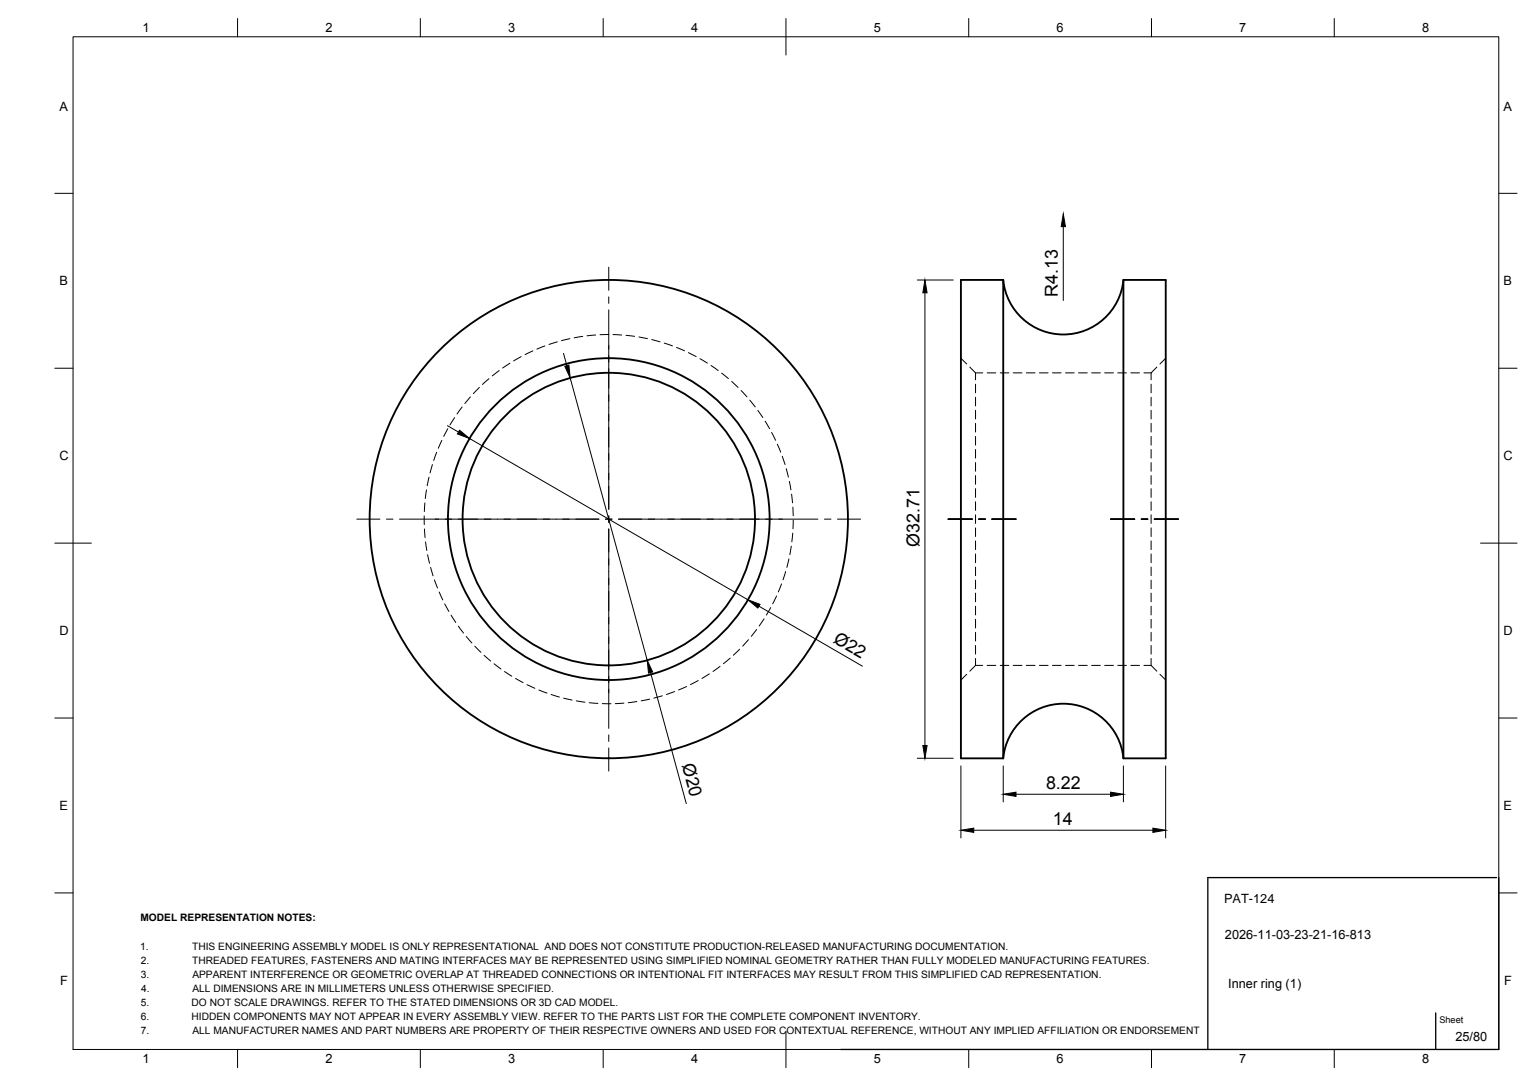
ISO-10303-21;
HEADER;
/* Generated by software containing ST-Developer
 * from STEP Tools, Inc. (www.steptools.com) 
 */

FILE_DESCRIPTION(
/* description */ ('XY cross-slide table'),
/* implementation_level */ '2;1');

FILE_NAME(
/* name */ 'Inner ring (1).step',
/* time_stamp */ '2026-10-28T03:22:46-07:00',
/* author */ (''),
/* organization */ (''),
/* preprocessor_version */ 'ST-DEVELOPER v20.2',
/* originating_system */ 'Autodesk Translation Framework v15.17.0.0',
/* authorisation */ '');

FILE_SCHEMA (('AUTOMOTIVE_DESIGN { 1 0 10303 214 3 1 1 }'));
ENDSEC;

DATA;
#10=MECHANICAL_DESIGN_GEOMETRIC_PRESENTATION_REPRESENTATION('',(#1693),#62984);
#1445=CONICAL_SURFACE('',#24426,1.05,0.785398163397449);
#1446=CONICAL_SURFACE('',#24433,1.05,0.785398163397449);
#1498=TOROIDAL_SURFACE('',#24415,1.675,0.412776);
#1520=SHAPE_REPRESENTATION_RELATIONSHIP('SRR','None',#63370,#1603);
#1603=ADVANCED_BREP_SHAPE_REPRESENTATION('',(#1806),#62907);
#1693=STYLED_ITEM('',(#63912),#1806);
#1806=MANIFOLD_SOLID_BREP('Body1',#22987);
#1992=FACE_BOUND('',#4488,.T.);
#1993=FACE_BOUND('',#4491,.T.);
#2397=PLANE('',#24428);
#2398=PLANE('',#24431);
#3064=FACE_OUTER_BOUND('',#4483,.T.);
#3065=FACE_OUTER_BOUND('',#4484,.T.);
#3066=FACE_OUTER_BOUND('',#4485,.T.);
#3067=FACE_OUTER_BOUND('',#4486,.T.);
#3068=FACE_OUTER_BOUND('',#4487,.T.);
#3069=FACE_OUTER_BOUND('',#4489,.T.);
#3070=FACE_OUTER_BOUND('',#4490,.T.);
#3071=FACE_OUTER_BOUND('',#4492,.T.);
#4483=EDGE_LOOP('',(#15752,#15753,#15754,#15755,#15756,#15757));
#4484=EDGE_LOOP('',(#15758,#15759,#15760,#15761,#15762));
#4485=EDGE_LOOP('',(#15763,#15764,#15765,#15766));
#4486=EDGE_LOOP('',(#15767,#15768,#15769,#15770));
#4487=EDGE_LOOP('',(#15771));
#4488=EDGE_LOOP('',(#15772));
#4489=EDGE_LOOP('',(#15773,#15774,#15775,#15776,#15777));
#4490=EDGE_LOOP('',(#15778));
#4491=EDGE_LOOP('',(#15779));
#4492=EDGE_LOOP('',(#15780,#15781,#15782,#15783));
#6123=LINE('',#34110,#7610);
#6124=LINE('',#34116,#7611);
#6125=LINE('',#34120,#7612);
#6126=LINE('',#34126,#7613);
#6127=LINE('',#34131,#7614);
#7610=VECTOR('',#27522,1.63531);
#7611=VECTOR('',#27529,1.);
#7612=VECTOR('',#27534,1.05);
#7613=VECTOR('',#27543,1.63531);
#7614=VECTOR('',#27550,1.05);
#9073=CIRCLE('',#24416,1.63531);
#9074=CIRCLE('',#24417,1.63531);
#9075=CIRCLE('',#24418,0.412776);
#9076=CIRCLE('',#24419,1.63531);
#9077=CIRCLE('',#24420,1.63531);
#9078=CIRCLE('',#24422,1.63531);
#9079=CIRCLE('',#24424,1.);
#9080=CIRCLE('',#24425,1.);
#9081=CIRCLE('',#24427,1.1);
#9082=CIRCLE('',#24430,1.63531);
#9083=CIRCLE('',#24432,1.1);
#10061=VERTEX_POINT('',#34099);
#10062=VERTEX_POINT('',#34100);
#10063=VERTEX_POINT('',#34103);
#10064=VERTEX_POINT('',#34105);
#10065=VERTEX_POINT('',#34109);
#10066=VERTEX_POINT('',#34113);
#10067=VERTEX_POINT('',#34115);
#10068=VERTEX_POINT('',#34119);
#10069=VERTEX_POINT('',#34124);
#10070=VERTEX_POINT('',#34128);
#12260=EDGE_CURVE('',#10061,#10062,#9073,.T.);
#12261=EDGE_CURVE('',#10062,#10061,#9074,.T.);
#12262=EDGE_CURVE('',#10062,#10063,#9075,.T.);
#12263=EDGE_CURVE('',#10064,#10063,#9076,.T.);
#12264=EDGE_CURVE('',#10063,#10064,#9077,.T.);
#12265=EDGE_CURVE('',#10064,#10065,#6123,.T.);
#12266=EDGE_CURVE('',#10065,#10065,#9078,.T.);
#12267=EDGE_CURVE('',#10066,#10066,#9079,.T.);
#12268=EDGE_CURVE('',#10066,#10067,#6124,.T.);
#12269=EDGE_CURVE('',#10067,#10067,#9080,.T.);
#12270=EDGE_CURVE('',#10067,#10068,#6125,.T.);
#12271=EDGE_CURVE('',#10068,#10068,#9081,.T.);
#12272=EDGE_CURVE('',#10069,#10069,#9082,.T.);
#12273=EDGE_CURVE('',#10069,#10061,#6126,.T.);
#12274=EDGE_CURVE('',#10070,#10070,#9083,.T.);
#12275=EDGE_CURVE('',#10070,#10066,#6127,.T.);
#15752=ORIENTED_EDGE('',*,*,#12260,.F.);
#15753=ORIENTED_EDGE('',*,*,#12261,.F.);
#15754=ORIENTED_EDGE('',*,*,#12262,.T.);
#15755=ORIENTED_EDGE('',*,*,#12263,.F.);
#15756=ORIENTED_EDGE('',*,*,#12264,.F.);
#15757=ORIENTED_EDGE('',*,*,#12262,.F.);
#15758=ORIENTED_EDGE('',*,*,#12263,.T.);
#15759=ORIENTED_EDGE('',*,*,#12264,.T.);
#15760=ORIENTED_EDGE('',*,*,#12265,.T.);
#15761=ORIENTED_EDGE('',*,*,#12266,.T.);
#15762=ORIENTED_EDGE('',*,*,#12265,.F.);
#15763=ORIENTED_EDGE('',*,*,#12267,.T.);
#15764=ORIENTED_EDGE('',*,*,#12268,.T.);
#15765=ORIENTED_EDGE('',*,*,#12269,.F.);
#15766=ORIENTED_EDGE('',*,*,#12268,.F.);
#15767=ORIENTED_EDGE('',*,*,#12269,.T.);
#15768=ORIENTED_EDGE('',*,*,#12270,.T.);
#15769=ORIENTED_EDGE('',*,*,#12271,.F.);
#15770=ORIENTED_EDGE('',*,*,#12270,.F.);
#15771=ORIENTED_EDGE('',*,*,#12266,.F.);
#15772=ORIENTED_EDGE('',*,*,#12271,.T.);
#15773=ORIENTED_EDGE('',*,*,#12272,.F.);
#15774=ORIENTED_EDGE('',*,*,#12273,.T.);
#15775=ORIENTED_EDGE('',*,*,#12260,.T.);
#15776=ORIENTED_EDGE('',*,*,#12261,.T.);
#15777=ORIENTED_EDGE('',*,*,#12273,.F.);
#15778=ORIENTED_EDGE('',*,*,#12272,.T.);
#15779=ORIENTED_EDGE('',*,*,#12274,.F.);
#15780=ORIENTED_EDGE('',*,*,#12274,.T.);
#15781=ORIENTED_EDGE('',*,*,#12275,.T.);
#15782=ORIENTED_EDGE('',*,*,#12267,.F.);
#15783=ORIENTED_EDGE('',*,*,#12275,.F.);
#21114=CYLINDRICAL_SURFACE('',#24421,1.63531);
#21115=CYLINDRICAL_SURFACE('',#24423,1.);
#21116=CYLINDRICAL_SURFACE('',#24429,1.63531);
#21845=ADVANCED_FACE('',(#3064),#1498,.F.);
#21846=ADVANCED_FACE('',(#3065),#21114,.T.);
#21847=ADVANCED_FACE('',(#3066),#21115,.F.);
#21848=ADVANCED_FACE('',(#3067),#1445,.F.);
#21849=ADVANCED_FACE('',(#3068,#1992),#2397,.T.);
#21850=ADVANCED_FACE('',(#3069),#21116,.T.);
#21851=ADVANCED_FACE('',(#3070,#1993),#2398,.T.);
#21852=ADVANCED_FACE('',(#3071),#1446,.F.);
#22987=CLOSED_SHELL('',(#21845,#21846,#21847,#21848,#21849,#21850,#21851,
#21852));
#24414=AXIS2_PLACEMENT_3D('',#34097,#27506,#27507);
#24415=AXIS2_PLACEMENT_3D('',#34098,#27508,#27509);
#24416=AXIS2_PLACEMENT_3D('',#34101,#27510,#27511);
#24417=AXIS2_PLACEMENT_3D('',#34102,#27512,#27513);
#24418=AXIS2_PLACEMENT_3D('',#34104,#27514,#27515);
#24419=AXIS2_PLACEMENT_3D('',#34106,#27516,#27517);
#24420=AXIS2_PLACEMENT_3D('',#34107,#27518,#27519);
#24421=AXIS2_PLACEMENT_3D('',#34108,#27520,#27521);
#24422=AXIS2_PLACEMENT_3D('',#34111,#27523,#27524);
#24423=AXIS2_PLACEMENT_3D('',#34112,#27525,#27526);
#24424=AXIS2_PLACEMENT_3D('',#34114,#27527,#27528);
#24425=AXIS2_PLACEMENT_3D('',#34117,#27530,#27531);
#24426=AXIS2_PLACEMENT_3D('',#34118,#27532,#27533);
#24427=AXIS2_PLACEMENT_3D('',#34121,#27535,#27536);
#24428=AXIS2_PLACEMENT_3D('',#34122,#27537,#27538);
#24429=AXIS2_PLACEMENT_3D('',#34123,#27539,#27540);
#24430=AXIS2_PLACEMENT_3D('',#34125,#27541,#27542);
#24431=AXIS2_PLACEMENT_3D('',#34127,#27544,#27545);
#24432=AXIS2_PLACEMENT_3D('',#34129,#27546,#27547);
#24433=AXIS2_PLACEMENT_3D('',#34130,#27548,#27549);
#27506=DIRECTION('axis',(0.,0.,1.));
#27507=DIRECTION('refdir',(1.,0.,0.));
#27508=DIRECTION('center_axis',(0.,-1.,0.));
#27509=DIRECTION('ref_axis',(0.,0.,-1.));
#27510=DIRECTION('center_axis',(0.,-1.,0.));
#27511=DIRECTION('ref_axis',(1.,0.,0.));
#27512=DIRECTION('center_axis',(0.,-1.,0.));
#27513=DIRECTION('ref_axis',(1.,0.,0.));
#27514=DIRECTION('center_axis',(1.,0.,1.22464679914735E-16));
#27515=DIRECTION('ref_axis',(-1.22464679914735E-16,0.,1.));
#27516=DIRECTION('center_axis',(0.,1.,0.));
#27517=DIRECTION('ref_axis',(1.,0.,0.));
#27518=DIRECTION('center_axis',(0.,1.,0.));
#27519=DIRECTION('ref_axis',(1.,0.,0.));
#27520=DIRECTION('center_axis',(0.,-1.,0.));
#27521=DIRECTION('ref_axis',(1.,0.,0.));
#27522=DIRECTION('',(0.,1.,0.));
#27523=DIRECTION('center_axis',(0.,-1.,0.));
#27524=DIRECTION('ref_axis',(1.,0.,0.));
#27525=DIRECTION('center_axis',(0.,-1.,0.));
#27526=DIRECTION('ref_axis',(1.,0.,0.));
#27527=DIRECTION('center_axis',(0.,-1.,0.));
#27528=DIRECTION('ref_axis',(1.,0.,0.));
#27529=DIRECTION('',(0.,1.,0.));
#27530=DIRECTION('center_axis',(0.,-1.,0.));
#27531=DIRECTION('ref_axis',(1.,0.,0.));
#27532=DIRECTION('center_axis',(0.,1.,0.));
#27533=DIRECTION('ref_axis',(1.,0.,0.));
#27534=DIRECTION('',(-0.707106781186548,0.707106781186547,-8.65956056235494E-17));
#27535=DIRECTION('center_axis',(0.,-1.,0.));
#27536=DIRECTION('ref_axis',(1.,0.,0.));
#27537=DIRECTION('center_axis',(0.,1.,0.));
#27538=DIRECTION('ref_axis',(0.,0.,1.));
#27539=DIRECTION('center_axis',(0.,-1.,0.));
#27540=DIRECTION('ref_axis',(1.,0.,0.));
#27541=DIRECTION('center_axis',(0.,-1.,0.));
#27542=DIRECTION('ref_axis',(1.,0.,0.));
#27543=DIRECTION('',(0.,1.,0.));
#27544=DIRECTION('center_axis',(0.,-1.,0.));
#27545=DIRECTION('ref_axis',(0.,0.,-1.));
#27546=DIRECTION('center_axis',(0.,-1.,0.));
#27547=DIRECTION('ref_axis',(1.,0.,0.));
#27548=DIRECTION('center_axis',(0.,-1.,0.));
#27549=DIRECTION('ref_axis',(1.,0.,0.));
#27550=DIRECTION('',(0.707106781186548,0.707106781186547,8.65956056235494E-17));
#34097=CARTESIAN_POINT('',(0.,0.,0.));
#34098=CARTESIAN_POINT('Origin',(0.,0.,0.));
#34099=CARTESIAN_POINT('',(-1.63531,-0.410863395882378,-2.00267715711366E-16));
#34100=CARTESIAN_POINT('',(-2.00267715711366E-16,-0.410863395882378,1.63531));
#34101=CARTESIAN_POINT('Origin',(0.,-0.410863395882378,0.));
#34102=CARTESIAN_POINT('Origin',(0.,-0.410863395882378,0.));
#34103=CARTESIAN_POINT('',(-2.00267715711366E-16,0.410863395882378,1.63531));
#34104=CARTESIAN_POINT('Origin',(-2.05128338857182E-16,0.,1.675));
#34105=CARTESIAN_POINT('',(-1.63531,0.410863395882378,2.00267715711366E-16));
#34106=CARTESIAN_POINT('Origin',(0.,0.410863395882378,0.));
#34107=CARTESIAN_POINT('Origin',(0.,0.410863395882378,0.));
#34108=CARTESIAN_POINT('Origin',(0.,0.,0.));
#34109=CARTESIAN_POINT('',(-1.63531,0.7,-2.00267715711366E-16));
#34110=CARTESIAN_POINT('',(-1.63531,0.,-2.00267715711366E-16));
#34111=CARTESIAN_POINT('Origin',(0.,0.7,0.));
#34112=CARTESIAN_POINT('Origin',(0.,0.,0.));
#34113=CARTESIAN_POINT('',(-1.,-0.6,-1.22464679914735E-16));
#34114=CARTESIAN_POINT('Origin',(0.,-0.6,0.));
#34115=CARTESIAN_POINT('',(-1.,0.6,-1.22464679914735E-16));
#34116=CARTESIAN_POINT('',(-1.,0.,-1.22464679914735E-16));
#34117=CARTESIAN_POINT('Origin',(0.,0.6,0.));
#34118=CARTESIAN_POINT('Origin',(0.,0.65,0.));
#34119=CARTESIAN_POINT('',(-1.1,0.7,-1.34711147906209E-16));
#34120=CARTESIAN_POINT('',(-1.05,0.65,-1.28587913910472E-16));
#34121=CARTESIAN_POINT('Origin',(0.,0.7,0.));
#34122=CARTESIAN_POINT('Origin',(1.63531,0.7,0.));
#34123=CARTESIAN_POINT('Origin',(0.,0.,0.));
#34124=CARTESIAN_POINT('',(-1.63531,-0.7,-2.00267715711366E-16));
#34125=CARTESIAN_POINT('Origin',(0.,-0.7,0.));
#34126=CARTESIAN_POINT('',(-1.63531,0.,-2.00267715711366E-16));
#34127=CARTESIAN_POINT('Origin',(1.1,-0.7,0.));
#34128=CARTESIAN_POINT('',(-1.1,-0.7,-1.34711147906209E-16));
#34129=CARTESIAN_POINT('Origin',(0.,-0.7,0.));
#34130=CARTESIAN_POINT('Origin',(0.,-0.65,0.));
#34131=CARTESIAN_POINT('',(-1.05,-0.65,-1.28587913910472E-16));
#62808=UNCERTAINTY_MEASURE_WITH_UNIT(LENGTH_MEASURE(0.001),#62985,
'DISTANCE_ACCURACY_VALUE',
'Maximum model space distance between geometric entities at asserted c
onnectivities');
#62885=UNCERTAINTY_MEASURE_WITH_UNIT(LENGTH_MEASURE(0.001),#62985,
'DISTANCE_ACCURACY_VALUE',
'Maximum model space distance between geometric entities at asserted c
onnectivities');
#62907=(
GEOMETRIC_REPRESENTATION_CONTEXT(3)
GLOBAL_UNCERTAINTY_ASSIGNED_CONTEXT((#62808))
GLOBAL_UNIT_ASSIGNED_CONTEXT((#62985,#62987,#62988))
REPRESENTATION_CONTEXT('','3D')
);
#62984=(
GEOMETRIC_REPRESENTATION_CONTEXT(3)
GLOBAL_UNCERTAINTY_ASSIGNED_CONTEXT((#62885))
GLOBAL_UNIT_ASSIGNED_CONTEXT((#62985,#62987,#62988))
REPRESENTATION_CONTEXT('','3D')
);
#62985=(
LENGTH_UNIT()
NAMED_UNIT(*)
SI_UNIT(.CENTI.,.METRE.)
);
#62987=(
NAMED_UNIT(*)
PLANE_ANGLE_UNIT()
SI_UNIT($,.RADIAN.)
);
#62988=(
NAMED_UNIT(*)
SI_UNIT($,.STERADIAN.)
SOLID_ANGLE_UNIT()
);
#63010=SHAPE_DEFINITION_REPRESENTATION(#63113,#63370);
#63113=PRODUCT_DEFINITION_SHAPE('',$,#63469);
#63370=SHAPE_REPRESENTATION('',(#24414),#62907);
#63447=PRODUCT_DEFINITION_CONTEXT('part definition',#63743,'design');
#63469=PRODUCT_DEFINITION('Inner ring (1)','Inner ring (1)',#63567,#63447);
#63567=PRODUCT_DEFINITION_FORMATION('',$,#63766);
#63743=APPLICATION_CONTEXT(
'Core Data for Automotive Mechanical Design Process');
#63744=PRODUCT_CONTEXT('part definition',#63743,'mechanical');
#63766=PRODUCT('Inner ring (1)','Inner ring (1)','Inner ring (1)',(#63744));
#63906=COLOUR_RGB('Grey',0.48,0.52,0.57);
#63907=FILL_AREA_STYLE_COLOUR('',#63906);
#63908=FILL_AREA_STYLE('',(#63907));
#63909=SURFACE_STYLE_FILL_AREA(#63908);
#63910=SURFACE_SIDE_STYLE('',(#63909));
#63911=SURFACE_STYLE_USAGE(.BOTH.,#63910);
#63912=PRESENTATION_STYLE_ASSIGNMENT((#63911));
ENDSEC;
END-ISO-10303-21;
